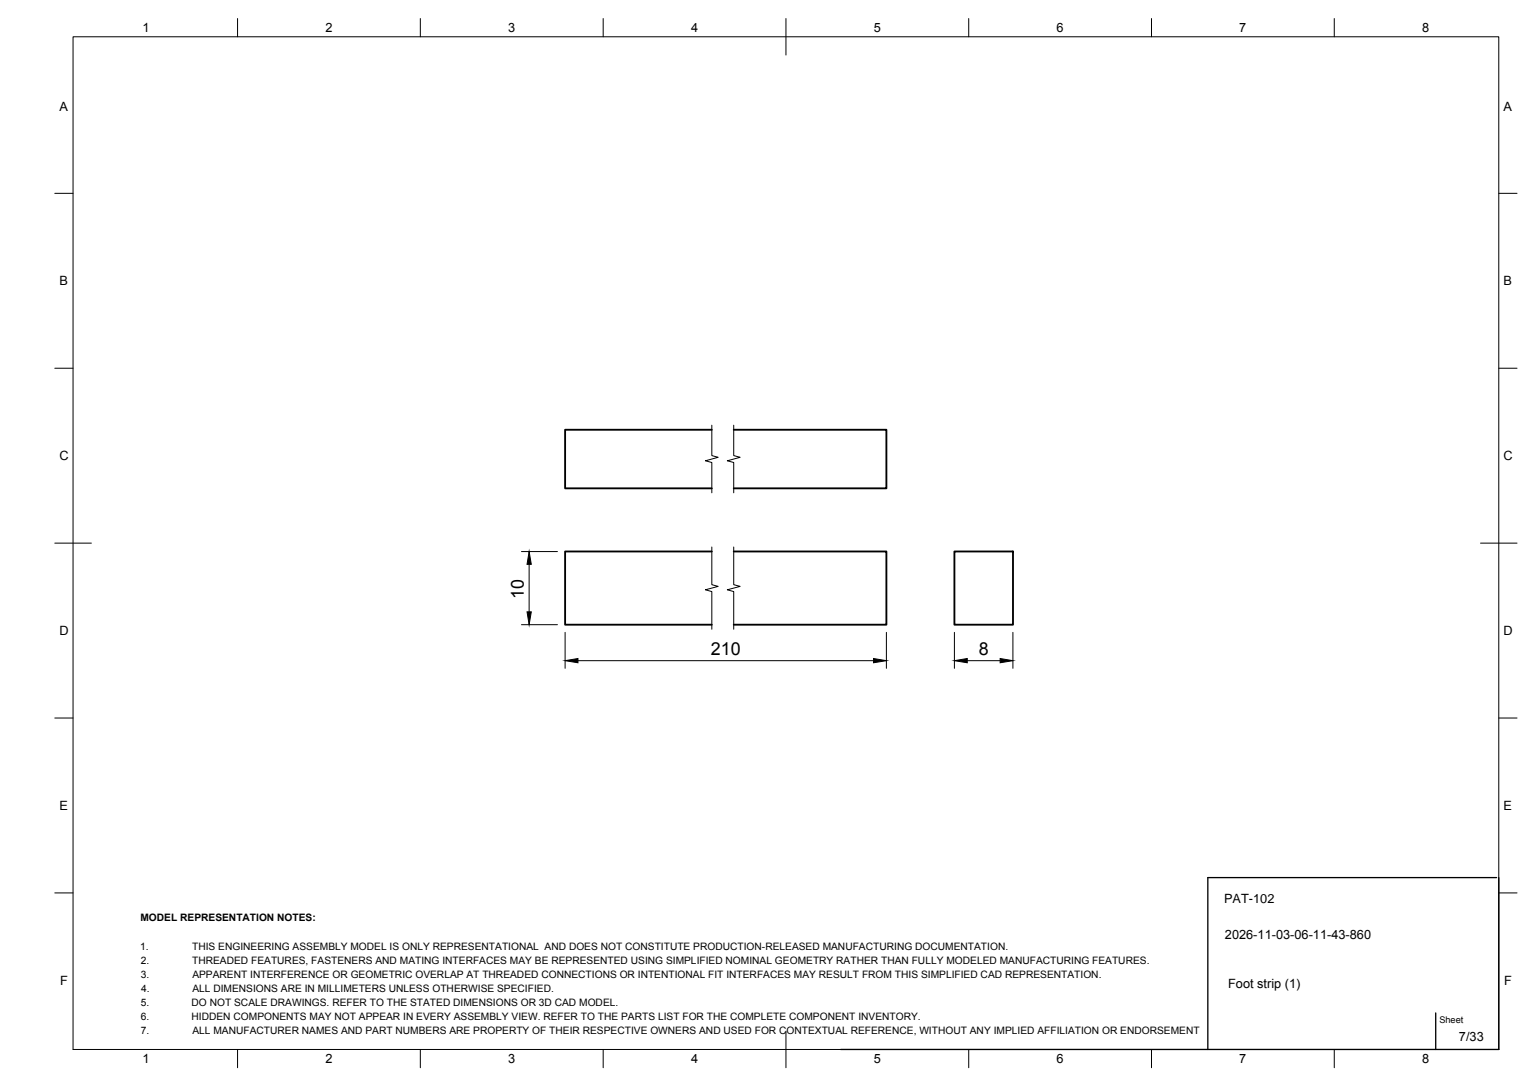
ISO-10303-21;
HEADER;
/* Generated by software containing ST-Developer
 * from STEP Tools, Inc. (www.steptools.com) 
 */

FILE_DESCRIPTION(
/* description */ ('Swing-away clamp arm'),
/* implementation_level */ '2;1');

FILE_NAME(
/* name */ 'Foot strip (1).step',
/* time_stamp */ '2026-10-28T03:26:03-07:00',
/* author */ (''),
/* organization */ (''),
/* preprocessor_version */ 'ST-DEVELOPER v20.2',
/* originating_system */ 'Autodesk Translation Framework v15.17.0.0',
/* authorisation */ '');

FILE_SCHEMA (('AUTOMOTIVE_DESIGN { 1 0 10303 214 3 1 1 }'));
ENDSEC;

DATA;
#10=MECHANICAL_DESIGN_GEOMETRIC_PRESENTATION_REPRESENTATION('',(#295),#10627);
#243=SHAPE_REPRESENTATION_RELATIONSHIP('SRR','None',#10741,#269);
#269=ADVANCED_BREP_SHAPE_REPRESENTATION('',(#329),#10600);
#295=STYLED_ITEM('',(#10951),#329);
#329=MANIFOLD_SOLID_BREP('Body1',#4901);
#470=PLANE('',#5252);
#471=PLANE('',#5253);
#472=PLANE('',#5254);
#473=PLANE('',#5255);
#474=PLANE('',#5256);
#475=PLANE('',#5257);
#653=FACE_OUTER_BOUND('',#968,.T.);
#654=FACE_OUTER_BOUND('',#969,.T.);
#655=FACE_OUTER_BOUND('',#970,.T.);
#656=FACE_OUTER_BOUND('',#971,.T.);
#657=FACE_OUTER_BOUND('',#972,.T.);
#658=FACE_OUTER_BOUND('',#973,.T.);
#968=EDGE_LOOP('',(#3353,#3354,#3355,#3356));
#969=EDGE_LOOP('',(#3357,#3358,#3359,#3360));
#970=EDGE_LOOP('',(#3361,#3362,#3363,#3364));
#971=EDGE_LOOP('',(#3365,#3366,#3367,#3368));
#972=EDGE_LOOP('',(#3369,#3370,#3371,#3372));
#973=EDGE_LOOP('',(#3373,#3374,#3375,#3376));
#1379=LINE('',#7570,#1701);
#1380=LINE('',#7572,#1702);
#1381=LINE('',#7574,#1703);
#1382=LINE('',#7575,#1704);
#1383=LINE('',#7578,#1705);
#1384=LINE('',#7580,#1706);
#1385=LINE('',#7581,#1707);
#1386=LINE('',#7584,#1708);
#1387=LINE('',#7586,#1709);
#1388=LINE('',#7587,#1710);
#1389=LINE('',#7589,#1711);
#1390=LINE('',#7590,#1712);
#1701=VECTOR('',#5958,1.);
#1702=VECTOR('',#5959,1.);
#1703=VECTOR('',#5960,1.);
#1704=VECTOR('',#5961,1.);
#1705=VECTOR('',#5964,1.);
#1706=VECTOR('',#5965,1.);
#1707=VECTOR('',#5966,1.);
#1708=VECTOR('',#5969,1.);
#1709=VECTOR('',#5970,1.);
#1710=VECTOR('',#5971,1.);
#1711=VECTOR('',#5974,1.);
#1712=VECTOR('',#5975,1.);
#2286=VERTEX_POINT('',#7568);
#2287=VERTEX_POINT('',#7569);
#2288=VERTEX_POINT('',#7571);
#2289=VERTEX_POINT('',#7573);
#2290=VERTEX_POINT('',#7577);
#2291=VERTEX_POINT('',#7579);
#2292=VERTEX_POINT('',#7583);
#2293=VERTEX_POINT('',#7585);
#2709=EDGE_CURVE('',#2286,#2287,#1379,.T.);
#2710=EDGE_CURVE('',#2287,#2288,#1380,.T.);
#2711=EDGE_CURVE('',#2289,#2288,#1381,.T.);
#2712=EDGE_CURVE('',#2286,#2289,#1382,.T.);
#2713=EDGE_CURVE('',#2290,#2286,#1383,.T.);
#2714=EDGE_CURVE('',#2291,#2289,#1384,.T.);
#2715=EDGE_CURVE('',#2290,#2291,#1385,.T.);
#2716=EDGE_CURVE('',#2292,#2290,#1386,.T.);
#2717=EDGE_CURVE('',#2293,#2291,#1387,.T.);
#2718=EDGE_CURVE('',#2292,#2293,#1388,.T.);
#2719=EDGE_CURVE('',#2287,#2292,#1389,.T.);
#2720=EDGE_CURVE('',#2288,#2293,#1390,.T.);
#3353=ORIENTED_EDGE('',*,*,#2709,.T.);
#3354=ORIENTED_EDGE('',*,*,#2710,.T.);
#3355=ORIENTED_EDGE('',*,*,#2711,.F.);
#3356=ORIENTED_EDGE('',*,*,#2712,.F.);
#3357=ORIENTED_EDGE('',*,*,#2713,.T.);
#3358=ORIENTED_EDGE('',*,*,#2712,.T.);
#3359=ORIENTED_EDGE('',*,*,#2714,.F.);
#3360=ORIENTED_EDGE('',*,*,#2715,.F.);
#3361=ORIENTED_EDGE('',*,*,#2716,.T.);
#3362=ORIENTED_EDGE('',*,*,#2715,.T.);
#3363=ORIENTED_EDGE('',*,*,#2717,.F.);
#3364=ORIENTED_EDGE('',*,*,#2718,.F.);
#3365=ORIENTED_EDGE('',*,*,#2719,.T.);
#3366=ORIENTED_EDGE('',*,*,#2718,.T.);
#3367=ORIENTED_EDGE('',*,*,#2720,.F.);
#3368=ORIENTED_EDGE('',*,*,#2710,.F.);
#3369=ORIENTED_EDGE('',*,*,#2720,.T.);
#3370=ORIENTED_EDGE('',*,*,#2717,.T.);
#3371=ORIENTED_EDGE('',*,*,#2714,.T.);
#3372=ORIENTED_EDGE('',*,*,#2711,.T.);
#3373=ORIENTED_EDGE('',*,*,#2719,.F.);
#3374=ORIENTED_EDGE('',*,*,#2709,.F.);
#3375=ORIENTED_EDGE('',*,*,#2713,.F.);
#3376=ORIENTED_EDGE('',*,*,#2716,.F.);
#4608=ADVANCED_FACE('',(#653),#470,.T.);
#4609=ADVANCED_FACE('',(#654),#471,.T.);
#4610=ADVANCED_FACE('',(#655),#472,.T.);
#4611=ADVANCED_FACE('',(#656),#473,.T.);
#4612=ADVANCED_FACE('',(#657),#474,.T.);
#4613=ADVANCED_FACE('',(#658),#475,.F.);
#4901=CLOSED_SHELL('',(#4608,#4609,#4610,#4611,#4612,#4613));
#5251=AXIS2_PLACEMENT_3D('',#7566,#5954,#5955);
#5252=AXIS2_PLACEMENT_3D('',#7567,#5956,#5957);
#5253=AXIS2_PLACEMENT_3D('',#7576,#5962,#5963);
#5254=AXIS2_PLACEMENT_3D('',#7582,#5967,#5968);
#5255=AXIS2_PLACEMENT_3D('',#7588,#5972,#5973);
#5256=AXIS2_PLACEMENT_3D('',#7591,#5976,#5977);
#5257=AXIS2_PLACEMENT_3D('',#7592,#5978,#5979);
#5954=DIRECTION('axis',(0.,0.,1.));
#5955=DIRECTION('refdir',(1.,0.,0.));
#5956=DIRECTION('center_axis',(0.,1.,0.));
#5957=DIRECTION('ref_axis',(-1.,0.,0.));
#5958=DIRECTION('',(-1.,0.,0.));
#5959=DIRECTION('',(0.,0.,1.));
#5960=DIRECTION('',(-1.,0.,0.));
#5961=DIRECTION('',(0.,0.,1.));
#5962=DIRECTION('center_axis',(1.,0.,0.));
#5963=DIRECTION('ref_axis',(0.,1.,0.));
#5964=DIRECTION('',(0.,1.,0.));
#5965=DIRECTION('',(0.,1.,0.));
#5966=DIRECTION('',(0.,0.,1.));
#5967=DIRECTION('center_axis',(0.,-1.,0.));
#5968=DIRECTION('ref_axis',(1.,0.,0.));
#5969=DIRECTION('',(1.,0.,0.));
#5970=DIRECTION('',(1.,0.,0.));
#5971=DIRECTION('',(0.,0.,1.));
#5972=DIRECTION('center_axis',(-1.,0.,0.));
#5973=DIRECTION('ref_axis',(0.,-1.,0.));
#5974=DIRECTION('',(0.,-1.,0.));
#5975=DIRECTION('',(0.,-1.,0.));
#5976=DIRECTION('center_axis',(0.,0.,1.));
#5977=DIRECTION('ref_axis',(1.,0.,0.));
#5978=DIRECTION('center_axis',(0.,0.,1.));
#5979=DIRECTION('ref_axis',(1.,0.,0.));
#7566=CARTESIAN_POINT('',(0.,0.,0.));
#7567=CARTESIAN_POINT('Origin',(16.,15.5,-0.8));
#7568=CARTESIAN_POINT('',(16.,15.5,-0.8));
#7569=CARTESIAN_POINT('',(15.,15.5,-0.8));
#7570=CARTESIAN_POINT('',(16.,15.5,-0.8));
#7571=CARTESIAN_POINT('',(15.,15.5,0.));
#7572=CARTESIAN_POINT('',(15.,15.5,-0.8));
#7573=CARTESIAN_POINT('',(16.,15.5,0.));
#7574=CARTESIAN_POINT('',(16.,15.5,0.));
#7575=CARTESIAN_POINT('',(16.,15.5,-0.8));
#7576=CARTESIAN_POINT('Origin',(16.,-5.5,-0.8));
#7577=CARTESIAN_POINT('',(16.,-5.5,-0.8));
#7578=CARTESIAN_POINT('',(16.,-5.5,-0.8));
#7579=CARTESIAN_POINT('',(16.,-5.5,0.));
#7580=CARTESIAN_POINT('',(16.,-5.5,0.));
#7581=CARTESIAN_POINT('',(16.,-5.5,-0.8));
#7582=CARTESIAN_POINT('Origin',(15.,-5.5,-0.8));
#7583=CARTESIAN_POINT('',(15.,-5.5,-0.8));
#7584=CARTESIAN_POINT('',(15.,-5.5,-0.8));
#7585=CARTESIAN_POINT('',(15.,-5.5,0.));
#7586=CARTESIAN_POINT('',(15.,-5.5,0.));
#7587=CARTESIAN_POINT('',(15.,-5.5,-0.8));
#7588=CARTESIAN_POINT('Origin',(15.,15.5,-0.8));
#7589=CARTESIAN_POINT('',(15.,15.5,-0.8));
#7590=CARTESIAN_POINT('',(15.,15.5,0.));
#7591=CARTESIAN_POINT('Origin',(15.5,5.,0.));
#7592=CARTESIAN_POINT('Origin',(15.5,5.,-0.8));
#10568=UNCERTAINTY_MEASURE_WITH_UNIT(LENGTH_MEASURE(0.001),#10628,
'DISTANCE_ACCURACY_VALUE',
'Maximum model space distance between geometric entities at asserted c
onnectivities');
#10595=UNCERTAINTY_MEASURE_WITH_UNIT(LENGTH_MEASURE(0.001),#10628,
'DISTANCE_ACCURACY_VALUE',
'Maximum model space distance between geometric entities at asserted c
onnectivities');
#10600=(
GEOMETRIC_REPRESENTATION_CONTEXT(3)
GLOBAL_UNCERTAINTY_ASSIGNED_CONTEXT((#10568))
GLOBAL_UNIT_ASSIGNED_CONTEXT((#10628,#10630,#10631))
REPRESENTATION_CONTEXT('','3D')
);
#10627=(
GEOMETRIC_REPRESENTATION_CONTEXT(3)
GLOBAL_UNCERTAINTY_ASSIGNED_CONTEXT((#10595))
GLOBAL_UNIT_ASSIGNED_CONTEXT((#10628,#10630,#10631))
REPRESENTATION_CONTEXT('','3D')
);
#10628=(
LENGTH_UNIT()
NAMED_UNIT(*)
SI_UNIT(.CENTI.,.METRE.)
);
#10630=(
NAMED_UNIT(*)
PLANE_ANGLE_UNIT()
SI_UNIT($,.RADIAN.)
);
#10631=(
NAMED_UNIT(*)
SI_UNIT($,.STERADIAN.)
SOLID_ANGLE_UNIT()
);
#10636=SHAPE_DEFINITION_REPRESENTATION(#10667,#10741);
#10667=PRODUCT_DEFINITION_SHAPE('',$,#10773);
#10741=SHAPE_REPRESENTATION('',(#5251),#10600);
#10768=PRODUCT_DEFINITION_CONTEXT('part definition',#10863,'design');
#10773=PRODUCT_DEFINITION('Foot strip (1)','Foot strip (1)',#10804,#10768);
#10804=PRODUCT_DEFINITION_FORMATION('',$,#10869);
#10863=APPLICATION_CONTEXT(
'Core Data for Automotive Mechanical Design Process');
#10864=PRODUCT_CONTEXT('part definition',#10863,'mechanical');
#10869=PRODUCT('Foot strip (1)','Foot strip (1)','Foot strip (1)',(#10864));
#10945=COLOUR_RGB('Light Blue',0.38,0.62,0.78);
#10946=FILL_AREA_STYLE_COLOUR('',#10945);
#10947=FILL_AREA_STYLE('',(#10946));
#10948=SURFACE_STYLE_FILL_AREA(#10947);
#10949=SURFACE_SIDE_STYLE('',(#10948));
#10950=SURFACE_STYLE_USAGE(.BOTH.,#10949);
#10951=PRESENTATION_STYLE_ASSIGNMENT((#10950));
ENDSEC;
END-ISO-10303-21;
